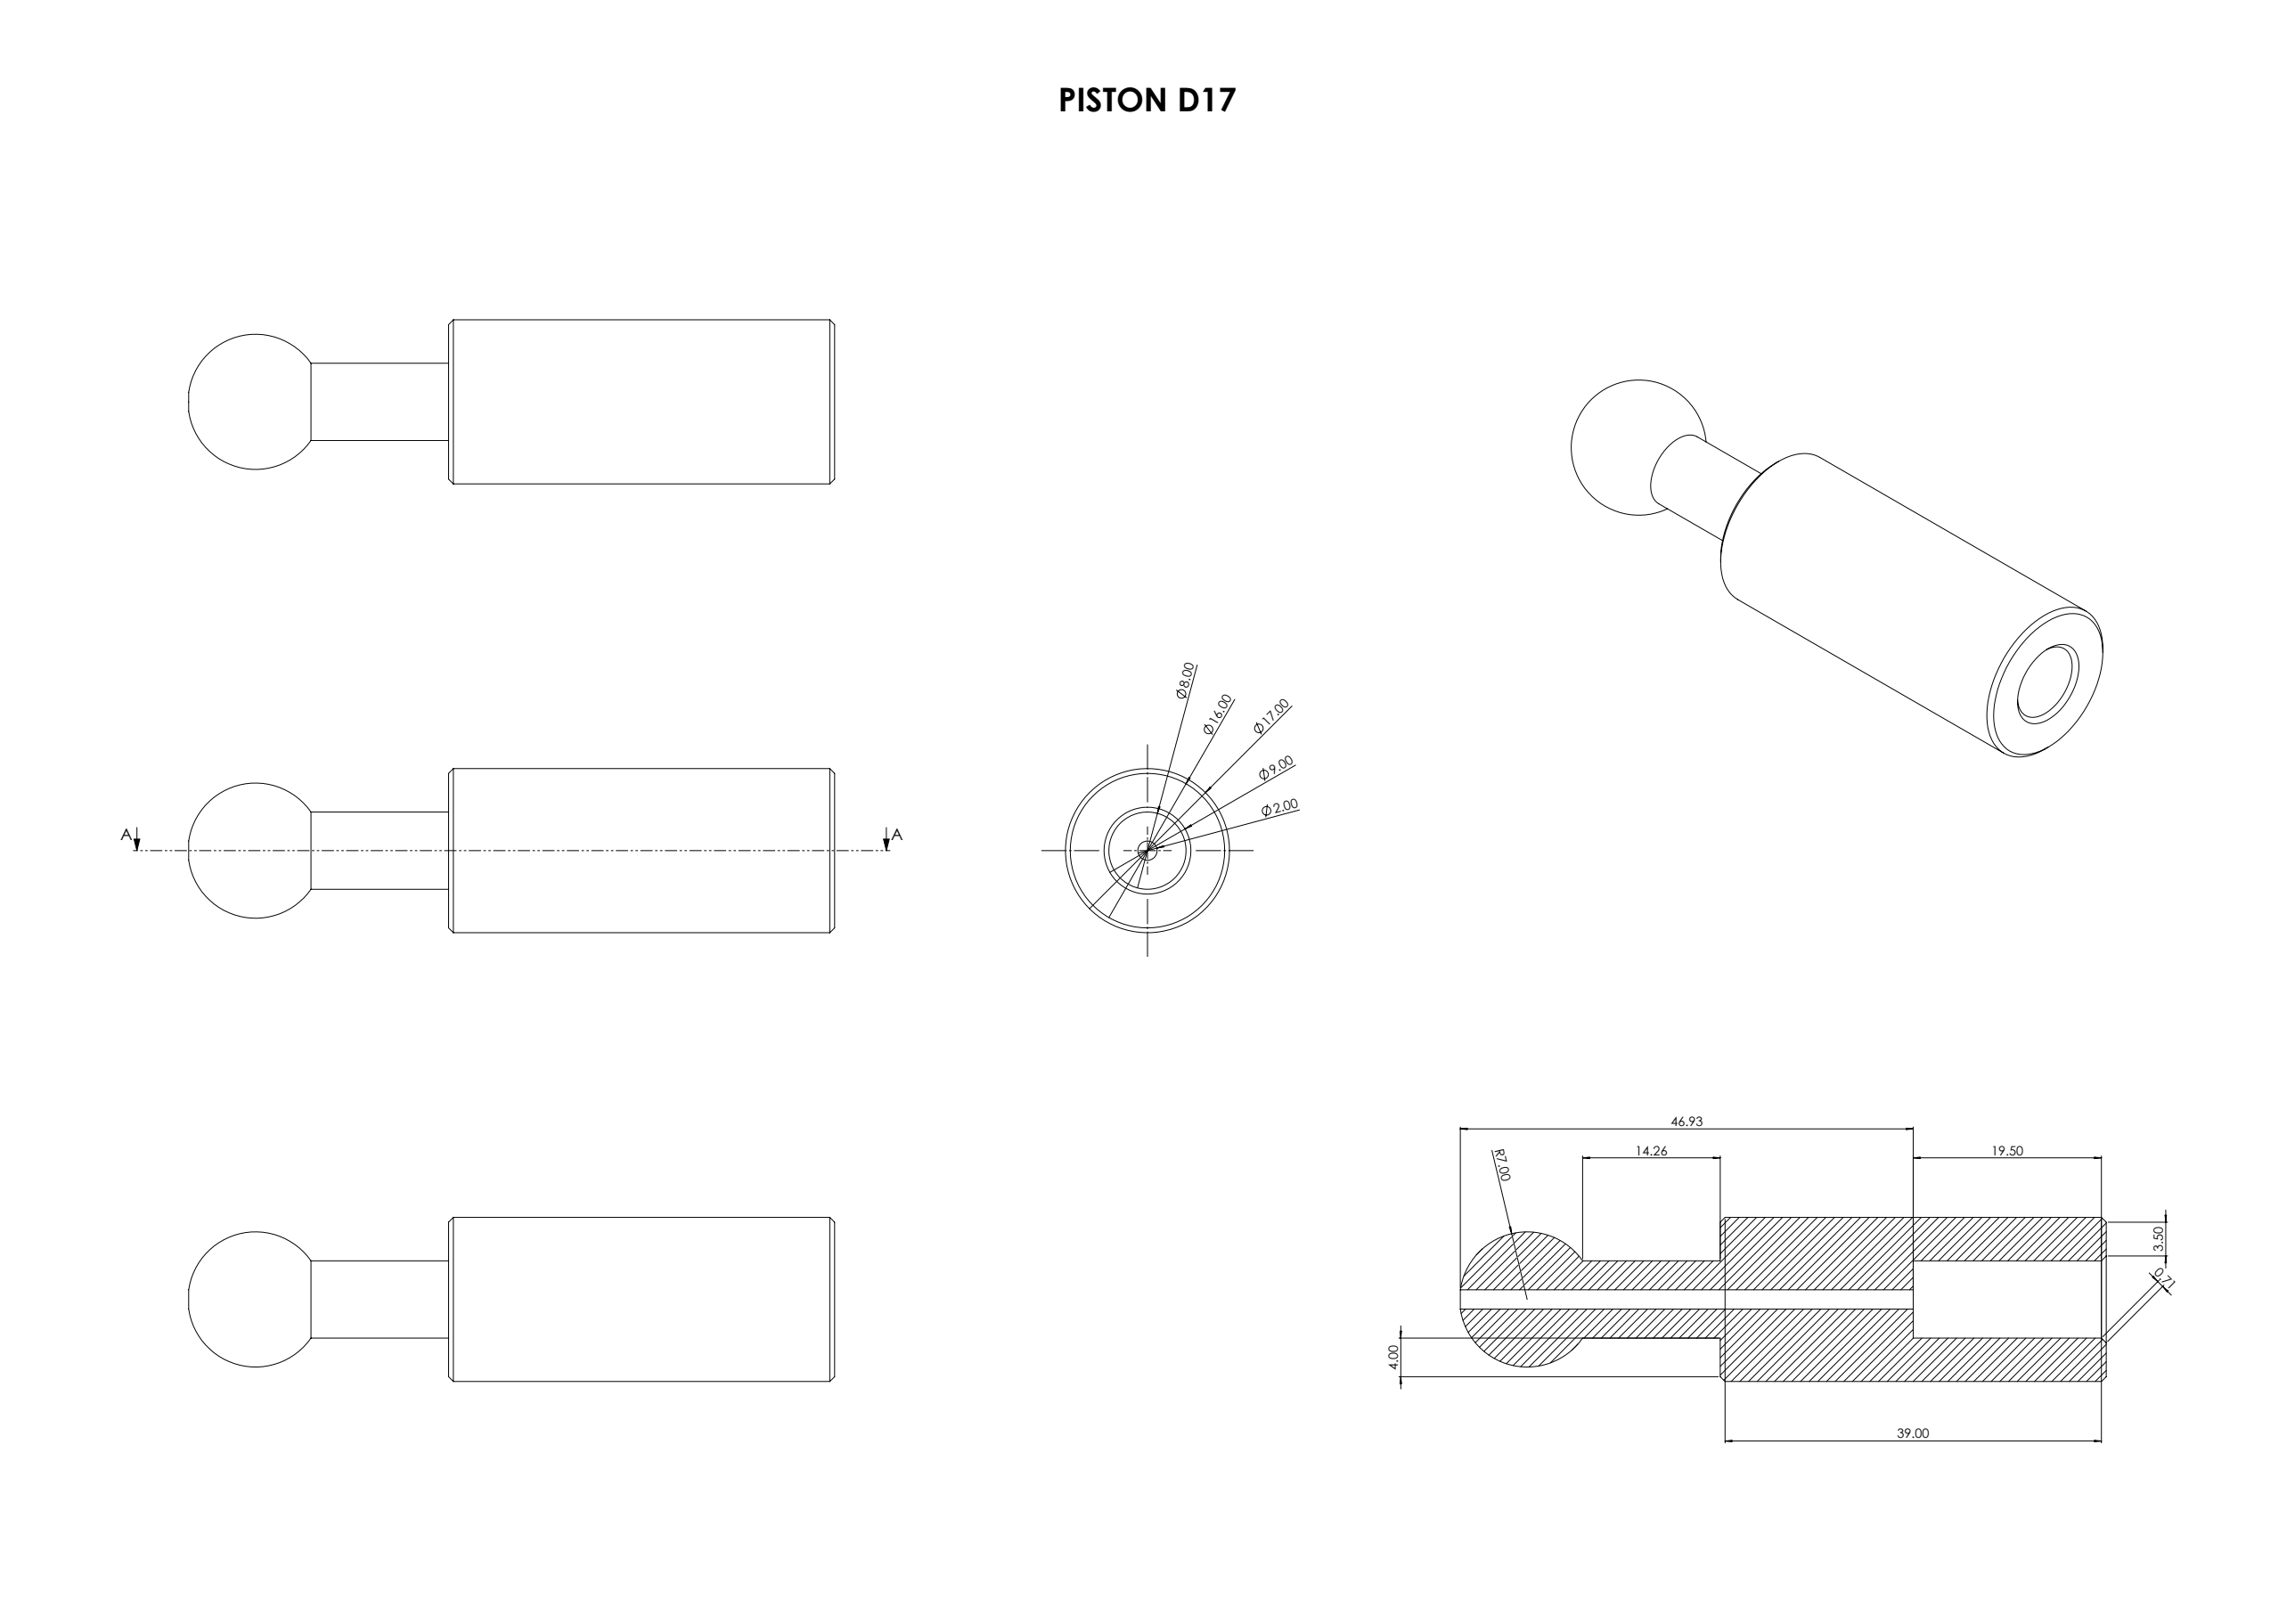
ISO-10303-21;
HEADER;
/* Generated by software containing ST-Developer
 * from STEP Tools, Inc. (www.steptools.com) 
 */

FILE_DESCRIPTION(
/* description */ (''),
/* implementation_level */ '2;1');

FILE_NAME(
/* name */ '05_Piston_D17.step',
/* time_stamp */ '2026-10-26T07:49:00-07:00',
/* author */ (''),
/* organization */ (''),
/* preprocessor_version */ 'ST-DEVELOPER v20.2',
/* originating_system */ 'Autodesk Translation Framework v15.15.0.0',
/* authorisation */ '');

FILE_SCHEMA (('AUTOMOTIVE_DESIGN { 1 0 10303 214 3 1 1 }'));
ENDSEC;

DATA;
#10=MECHANICAL_DESIGN_GEOMETRIC_PRESENTATION_REPRESENTATION('',(#187),#38507);
#131=(
BOUNDED_SURFACE()
B_SPLINE_SURFACE(2,2,((#27036,#27037,#27038,#27039,#27040,#27041,#27042,
#27043,#27044),(#27045,#27046,#27047,#27048,#27049,#27050,#27051,#27052,
#27053),(#27054,#27055,#27056,#27057,#27058,#27059,#27060,#27061,#27062),
(#27063,#27064,#27065,#27066,#27067,#27068,#27069,#27070,#27071),(#27072,
#27073,#27074,#27075,#27076,#27077,#27078,#27079,#27080)),.UNSPECIFIED.,
 .F.,.T.,.F.)
B_SPLINE_SURFACE_WITH_KNOTS((3,2,3),(3,2,2,2,3),(-1.42752879197468,-0.232447556257835,
0.962633679459007),(-3.14159265358979,-1.5707963267949,0.,1.5707963267949,
3.14159265358979),.UNSPECIFIED.)
GEOMETRIC_REPRESENTATION_ITEM()
RATIONAL_B_SPLINE_SURFACE(((1.,0.707106781186548,1.,0.707106781186548,1.,
0.707106781186548,1.,0.707106781186548,1.),(0.826721789080264,0.584580583213329,
0.826721789080264,0.584580583213329,0.826721789080264,0.584580583213329,
0.826721789080264,0.584580583213329,0.826721789080264),(1.,0.707106781186548,
1.,0.707106781186548,1.,0.707106781186548,1.,0.707106781186548,1.),(0.826721789080262,
0.584580583213328,0.826721789080262,0.584580583213328,0.826721789080262,
0.584580583213328,0.826721789080262,0.584580583213328,0.826721789080262),
(1.,0.707106781186548,1.,0.707106781186548,1.,0.707106781186548,1.,0.707106781186548,
1.)))
REPRESENTATION_ITEM('')
SURFACE()
);
#157=SHAPE_REPRESENTATION_RELATIONSHIP('SRR','None',#38585,#172);
#172=ADVANCED_BREP_SHAPE_REPRESENTATION('',(#202),#38502);
#187=STYLED_ITEM('',(#38713),#202);
#202=MANIFOLD_SOLID_BREP('Body1',#15081);
#507=FACE_BOUND('',#3150,.T.);
#508=FACE_BOUND('',#3153,.T.);
#509=FACE_BOUND('',#3156,.T.);
#802=PLANE('',#16260);
#803=PLANE('',#16266);
#804=PLANE('',#16271);
#1505=CYLINDRICAL_SURFACE('',#16258,4.);
#1506=CYLINDRICAL_SURFACE('',#16262,1.);
#1507=CYLINDRICAL_SURFACE('',#16267,4.);
#1508=CYLINDRICAL_SURFACE('',#16275,8.5);
#2170=FACE_OUTER_BOUND('',#3147,.T.);
#2171=FACE_OUTER_BOUND('',#3148,.T.);
#2172=FACE_OUTER_BOUND('',#3149,.T.);
#2173=FACE_OUTER_BOUND('',#3151,.T.);
#2174=FACE_OUTER_BOUND('',#3152,.T.);
#2175=FACE_OUTER_BOUND('',#3154,.T.);
#2176=FACE_OUTER_BOUND('',#3155,.T.);
#2177=FACE_OUTER_BOUND('',#3157,.T.);
#2178=FACE_OUTER_BOUND('',#3158,.T.);
#2179=FACE_OUTER_BOUND('',#3159,.T.);
#2180=FACE_OUTER_BOUND('',#3160,.T.);
#3147=EDGE_LOOP('',(#12485,#12486,#12487,#12488));
#3148=EDGE_LOOP('',(#12489,#12490,#12491,#12492));
#3149=EDGE_LOOP('',(#12493));
#3150=EDGE_LOOP('',(#12494));
#3151=EDGE_LOOP('',(#12495,#12496,#12497,#12498,#12499));
#3152=EDGE_LOOP('',(#12500));
#3153=EDGE_LOOP('',(#12501));
#3154=EDGE_LOOP('',(#12502,#12503,#12504,#12505,#12506));
#3155=EDGE_LOOP('',(#12507));
#3156=EDGE_LOOP('',(#12508));
#3157=EDGE_LOOP('',(#12509,#12510,#12511,#12512));
#3158=EDGE_LOOP('',(#12513,#12514,#12515,#12516));
#3159=EDGE_LOOP('',(#12517,#12518,#12519,#12520));
#3160=EDGE_LOOP('',(#12521,#12522,#12523,#12524,#12525,#12526));
#4129=LINE('',#26997,#5198);
#4130=LINE('',#27002,#5199);
#4131=LINE('',#27011,#5200);
#4132=LINE('',#27019,#5201);
#4133=LINE('',#27029,#5202);
#4134=LINE('',#27033,#5203);
#4135=LINE('',#27035,#5204);
#5198=VECTOR('',#19382,4.25);
#5199=VECTOR('',#19389,4.);
#5200=VECTOR('',#19398,1.);
#5201=VECTOR('',#19409,4.);
#5202=VECTOR('',#19422,8.25);
#5203=VECTOR('',#19427,8.5);
#5204=VECTOR('',#19430,8.25);
#6114=CIRCLE('',#16256,4.5);
#6115=CIRCLE('',#16257,4.);
#6116=CIRCLE('',#16259,4.);
#6117=CIRCLE('',#16261,8.);
#6118=CIRCLE('',#16263,1.);
#6119=CIRCLE('',#16264,1.);
#6120=CIRCLE('',#16265,1.);
#6121=CIRCLE('',#16268,4.);
#6122=CIRCLE('',#16269,4.);
#6123=CIRCLE('',#16270,4.);
#6124=CIRCLE('',#16272,8.);
#6125=CIRCLE('',#16274,8.5);
#6126=CIRCLE('',#16276,8.5);
#6127=CIRCLE('',#16278,6.99981782686978);
#7119=VERTEX_POINT('',#26994);
#7120=VERTEX_POINT('',#26996);
#7121=VERTEX_POINT('',#27000);
#7122=VERTEX_POINT('',#27004);
#7123=VERTEX_POINT('',#27007);
#7124=VERTEX_POINT('',#27008);
#7125=VERTEX_POINT('',#27010);
#7126=VERTEX_POINT('',#27016);
#7127=VERTEX_POINT('',#27018);
#7128=VERTEX_POINT('',#27020);
#7129=VERTEX_POINT('',#27024);
#7130=VERTEX_POINT('',#27027);
#7131=VERTEX_POINT('',#27031);
#8991=EDGE_CURVE('',#7119,#7119,#6114,.T.);
#8992=EDGE_CURVE('',#7119,#7120,#4129,.T.);
#8993=EDGE_CURVE('',#7120,#7120,#6115,.T.);
#8994=EDGE_CURVE('',#7121,#7121,#6116,.T.);
#8995=EDGE_CURVE('',#7121,#7120,#4130,.T.);
#8996=EDGE_CURVE('',#7122,#7122,#6117,.T.);
#8997=EDGE_CURVE('',#7123,#7124,#6118,.T.);
#8998=EDGE_CURVE('',#7123,#7125,#4131,.T.);
#8999=EDGE_CURVE('',#7125,#7125,#6119,.T.);
#9000=EDGE_CURVE('',#7124,#7123,#6120,.T.);
#9001=EDGE_CURVE('',#7126,#7126,#6121,.T.);
#9002=EDGE_CURVE('',#7126,#7127,#4132,.T.);
#9003=EDGE_CURVE('',#7127,#7128,#6122,.T.);
#9004=EDGE_CURVE('',#7128,#7127,#6123,.T.);
#9005=EDGE_CURVE('',#7129,#7129,#6124,.T.);
#9006=EDGE_CURVE('',#7130,#7130,#6125,.T.);
#9007=EDGE_CURVE('',#7130,#7129,#4133,.T.);
#9008=EDGE_CURVE('',#7131,#7131,#6126,.T.);
#9009=EDGE_CURVE('',#7131,#7130,#4134,.T.);
#9010=EDGE_CURVE('',#7122,#7131,#4135,.T.);
#9011=EDGE_CURVE('',#7128,#7124,#6127,.T.);
#12485=ORIENTED_EDGE('',*,*,#8991,.T.);
#12486=ORIENTED_EDGE('',*,*,#8992,.T.);
#12487=ORIENTED_EDGE('',*,*,#8993,.T.);
#12488=ORIENTED_EDGE('',*,*,#8992,.F.);
#12489=ORIENTED_EDGE('',*,*,#8994,.F.);
#12490=ORIENTED_EDGE('',*,*,#8995,.T.);
#12491=ORIENTED_EDGE('',*,*,#8993,.F.);
#12492=ORIENTED_EDGE('',*,*,#8995,.F.);
#12493=ORIENTED_EDGE('',*,*,#8996,.T.);
#12494=ORIENTED_EDGE('',*,*,#8991,.F.);
#12495=ORIENTED_EDGE('',*,*,#8997,.F.);
#12496=ORIENTED_EDGE('',*,*,#8998,.T.);
#12497=ORIENTED_EDGE('',*,*,#8999,.F.);
#12498=ORIENTED_EDGE('',*,*,#8998,.F.);
#12499=ORIENTED_EDGE('',*,*,#9000,.F.);
#12500=ORIENTED_EDGE('',*,*,#8994,.T.);
#12501=ORIENTED_EDGE('',*,*,#8999,.T.);
#12502=ORIENTED_EDGE('',*,*,#9001,.F.);
#12503=ORIENTED_EDGE('',*,*,#9002,.T.);
#12504=ORIENTED_EDGE('',*,*,#9003,.T.);
#12505=ORIENTED_EDGE('',*,*,#9004,.T.);
#12506=ORIENTED_EDGE('',*,*,#9002,.F.);
#12507=ORIENTED_EDGE('',*,*,#9005,.F.);
#12508=ORIENTED_EDGE('',*,*,#9001,.T.);
#12509=ORIENTED_EDGE('',*,*,#9006,.F.);
#12510=ORIENTED_EDGE('',*,*,#9007,.T.);
#12511=ORIENTED_EDGE('',*,*,#9005,.T.);
#12512=ORIENTED_EDGE('',*,*,#9007,.F.);
#12513=ORIENTED_EDGE('',*,*,#9008,.F.);
#12514=ORIENTED_EDGE('',*,*,#9009,.T.);
#12515=ORIENTED_EDGE('',*,*,#9006,.T.);
#12516=ORIENTED_EDGE('',*,*,#9009,.F.);
#12517=ORIENTED_EDGE('',*,*,#8996,.F.);
#12518=ORIENTED_EDGE('',*,*,#9010,.T.);
#12519=ORIENTED_EDGE('',*,*,#9008,.T.);
#12520=ORIENTED_EDGE('',*,*,#9010,.F.);
#12521=ORIENTED_EDGE('',*,*,#9003,.F.);
#12522=ORIENTED_EDGE('',*,*,#9004,.F.);
#12523=ORIENTED_EDGE('',*,*,#9011,.T.);
#12524=ORIENTED_EDGE('',*,*,#9000,.T.);
#12525=ORIENTED_EDGE('',*,*,#8997,.T.);
#12526=ORIENTED_EDGE('',*,*,#9011,.F.);
#14175=CONICAL_SURFACE('',#16255,4.25,0.78539816339745);
#14176=CONICAL_SURFACE('',#16273,8.25,0.78539816339745);
#14177=CONICAL_SURFACE('',#16277,8.25,0.78539816339745);
#14737=ADVANCED_FACE('',(#2170),#14175,.F.);
#14738=ADVANCED_FACE('',(#2171),#1505,.F.);
#14739=ADVANCED_FACE('',(#2172,#507),#802,.T.);
#14740=ADVANCED_FACE('',(#2173),#1506,.F.);
#14741=ADVANCED_FACE('',(#2174,#508),#803,.F.);
#14742=ADVANCED_FACE('',(#2175),#1507,.T.);
#14743=ADVANCED_FACE('',(#2176,#509),#804,.T.);
#14744=ADVANCED_FACE('',(#2177),#14176,.T.);
#14745=ADVANCED_FACE('',(#2178),#1508,.T.);
#14746=ADVANCED_FACE('',(#2179),#14177,.T.);
#14747=ADVANCED_FACE('',(#2180),#131,.F.);
#15081=CLOSED_SHELL('',(#14737,#14738,#14739,#14740,#14741,#14742,#14743,
#14744,#14745,#14746,#14747));
#16254=AXIS2_PLACEMENT_3D('',#26992,#19376,#19377);
#16255=AXIS2_PLACEMENT_3D('',#26993,#19378,#19379);
#16256=AXIS2_PLACEMENT_3D('',#26995,#19380,#19381);
#16257=AXIS2_PLACEMENT_3D('',#26998,#19383,#19384);
#16258=AXIS2_PLACEMENT_3D('',#26999,#19385,#19386);
#16259=AXIS2_PLACEMENT_3D('',#27001,#19387,#19388);
#16260=AXIS2_PLACEMENT_3D('',#27003,#19390,#19391);
#16261=AXIS2_PLACEMENT_3D('',#27005,#19392,#19393);
#16262=AXIS2_PLACEMENT_3D('',#27006,#19394,#19395);
#16263=AXIS2_PLACEMENT_3D('',#27009,#19396,#19397);
#16264=AXIS2_PLACEMENT_3D('',#27012,#19399,#19400);
#16265=AXIS2_PLACEMENT_3D('',#27013,#19401,#19402);
#16266=AXIS2_PLACEMENT_3D('',#27014,#19403,#19404);
#16267=AXIS2_PLACEMENT_3D('',#27015,#19405,#19406);
#16268=AXIS2_PLACEMENT_3D('',#27017,#19407,#19408);
#16269=AXIS2_PLACEMENT_3D('',#27021,#19410,#19411);
#16270=AXIS2_PLACEMENT_3D('',#27022,#19412,#19413);
#16271=AXIS2_PLACEMENT_3D('',#27023,#19414,#19415);
#16272=AXIS2_PLACEMENT_3D('',#27025,#19416,#19417);
#16273=AXIS2_PLACEMENT_3D('',#27026,#19418,#19419);
#16274=AXIS2_PLACEMENT_3D('',#27028,#19420,#19421);
#16275=AXIS2_PLACEMENT_3D('',#27030,#19423,#19424);
#16276=AXIS2_PLACEMENT_3D('',#27032,#19425,#19426);
#16277=AXIS2_PLACEMENT_3D('',#27034,#19428,#19429);
#16278=AXIS2_PLACEMENT_3D('',#27081,#19431,#19432);
#19376=DIRECTION('axis',(0.,0.,1.));
#19377=DIRECTION('refdir',(1.,0.,0.));
#19378=DIRECTION('center_axis',(1.,0.,0.));
#19379=DIRECTION('ref_axis',(0.,1.,0.));
#19380=DIRECTION('center_axis',(1.,0.,0.));
#19381=DIRECTION('ref_axis',(0.,1.,0.));
#19382=DIRECTION('',(-0.707106781186546,0.707106781186549,8.65956056235495E-17));
#19383=DIRECTION('center_axis',(-1.,0.,0.));
#19384=DIRECTION('ref_axis',(0.,1.,0.));
#19385=DIRECTION('center_axis',(1.,0.,0.));
#19386=DIRECTION('ref_axis',(0.,1.,0.));
#19387=DIRECTION('center_axis',(1.,0.,0.));
#19388=DIRECTION('ref_axis',(0.,0.,-1.));
#19389=DIRECTION('',(1.,0.,0.));
#19390=DIRECTION('center_axis',(1.,0.,0.));
#19391=DIRECTION('ref_axis',(0.,0.,-1.));
#19392=DIRECTION('center_axis',(1.,0.,0.));
#19393=DIRECTION('ref_axis',(0.,0.,-1.));
#19394=DIRECTION('center_axis',(1.,0.,0.));
#19395=DIRECTION('ref_axis',(0.,1.,0.));
#19396=DIRECTION('center_axis',(1.,0.,0.));
#19397=DIRECTION('ref_axis',(0.,1.,0.));
#19398=DIRECTION('',(1.,0.,0.));
#19399=DIRECTION('center_axis',(-1.,0.,0.));
#19400=DIRECTION('ref_axis',(0.,1.,0.));
#19401=DIRECTION('center_axis',(1.,0.,0.));
#19402=DIRECTION('ref_axis',(0.,1.,0.));
#19403=DIRECTION('center_axis',(-1.,0.,0.));
#19404=DIRECTION('ref_axis',(0.,0.,1.));
#19405=DIRECTION('center_axis',(1.,0.,0.));
#19406=DIRECTION('ref_axis',(0.,1.,0.));
#19407=DIRECTION('center_axis',(1.,0.,0.));
#19408=DIRECTION('ref_axis',(0.,0.,-1.));
#19409=DIRECTION('',(-1.,0.,0.));
#19410=DIRECTION('center_axis',(1.,0.,0.));
#19411=DIRECTION('ref_axis',(0.,0.,-1.));
#19412=DIRECTION('center_axis',(1.,0.,0.));
#19413=DIRECTION('ref_axis',(0.,0.,-1.));
#19414=DIRECTION('center_axis',(-1.,0.,0.));
#19415=DIRECTION('ref_axis',(0.,0.,1.));
#19416=DIRECTION('center_axis',(1.,0.,0.));
#19417=DIRECTION('ref_axis',(0.,0.,-1.));
#19418=DIRECTION('center_axis',(1.,0.,0.));
#19419=DIRECTION('ref_axis',(0.,1.,0.));
#19420=DIRECTION('center_axis',(1.,0.,0.));
#19421=DIRECTION('ref_axis',(0.,0.,-1.));
#19422=DIRECTION('',(-0.707106781186547,0.707106781186548,8.65956056235494E-17));
#19423=DIRECTION('center_axis',(1.,0.,0.));
#19424=DIRECTION('ref_axis',(0.,1.,0.));
#19425=DIRECTION('center_axis',(1.,0.,0.));
#19426=DIRECTION('ref_axis',(0.,0.,-1.));
#19427=DIRECTION('',(-1.,0.,0.));
#19428=DIRECTION('center_axis',(-1.,0.,0.));
#19429=DIRECTION('ref_axis',(0.,1.,0.));
#19430=DIRECTION('',(-0.707106781186547,-0.707106781186548,-8.65956056235494E-17));
#19431=DIRECTION('center_axis',(0.,-1.,-1.22464679914735E-16));
#19432=DIRECTION('ref_axis',(0.,-1.22464679914735E-16,1.));
#26992=CARTESIAN_POINT('',(0.,0.,0.));
#26993=CARTESIAN_POINT('Origin',(59.75,0.,0.));
#26994=CARTESIAN_POINT('',(60.,-4.5,-5.51091059616309E-16));
#26995=CARTESIAN_POINT('Origin',(60.,0.,0.));
#26996=CARTESIAN_POINT('',(59.5,-4.,4.89858719658941E-16));
#26997=CARTESIAN_POINT('',(59.75,-4.25,-5.20474889637625E-16));
#26998=CARTESIAN_POINT('Origin',(59.5,0.,0.));
#26999=CARTESIAN_POINT('Origin',(50.05,0.,0.));
#27000=CARTESIAN_POINT('',(40.,-4.,-4.89858719658941E-16));
#27001=CARTESIAN_POINT('Origin',(40.,0.,0.));
#27002=CARTESIAN_POINT('',(50.05,-4.,-4.89858719658941E-16));
#27003=CARTESIAN_POINT('Origin',(60.,0.,0.));
#27004=CARTESIAN_POINT('',(60.,-8.,-9.79717439317882E-16));
#27005=CARTESIAN_POINT('Origin',(60.,0.,0.));
#27006=CARTESIAN_POINT('Origin',(26.5,0.,0.));
#27007=CARTESIAN_POINT('',(-6.92828513265203,-1.,-1.22464679914735E-16));
#27008=CARTESIAN_POINT('',(-6.92828513265203,-1.22464679914735E-16,1.));
#27009=CARTESIAN_POINT('Origin',(-6.92828513265203,0.,0.));
#27010=CARTESIAN_POINT('',(40.,-1.,1.22464679914735E-16));
#27011=CARTESIAN_POINT('',(26.5,-1.,-1.22464679914735E-16));
#27012=CARTESIAN_POINT('Origin',(40.,0.,0.));
#27013=CARTESIAN_POINT('Origin',(-6.92828513265203,0.,0.));
#27014=CARTESIAN_POINT('Origin',(40.,4.,0.));
#27015=CARTESIAN_POINT('Origin',(12.872281323269,0.,0.));
#27016=CARTESIAN_POINT('',(20.,-4.,-4.89858719658941E-16));
#27017=CARTESIAN_POINT('Origin',(20.,0.,0.));
#27018=CARTESIAN_POINT('',(5.74456264653803,-4.,-4.89858719658941E-16));
#27019=CARTESIAN_POINT('',(12.872281323269,-4.,-4.89858719658941E-16));
#27020=CARTESIAN_POINT('',(5.74456264653803,-4.89858719658941E-16,4.));
#27021=CARTESIAN_POINT('Origin',(5.74456264653803,0.,0.));
#27022=CARTESIAN_POINT('Origin',(5.74456264653803,0.,0.));
#27023=CARTESIAN_POINT('Origin',(20.,8.,0.));
#27024=CARTESIAN_POINT('',(20.,-8.,-9.79717439317883E-16));
#27025=CARTESIAN_POINT('Origin',(20.,0.,0.));
#27026=CARTESIAN_POINT('Origin',(20.25,0.,0.));
#27027=CARTESIAN_POINT('',(20.5,-8.5,-1.04094977927525E-15));
#27028=CARTESIAN_POINT('Origin',(20.5,0.,0.));
#27029=CARTESIAN_POINT('',(20.25,-8.25,-1.01033360929657E-15));
#27030=CARTESIAN_POINT('Origin',(40.,0.,0.));
#27031=CARTESIAN_POINT('',(59.5,-8.5,-1.04094977927525E-15));
#27032=CARTESIAN_POINT('Origin',(59.5,0.,0.));
#27033=CARTESIAN_POINT('',(40.,-8.5,-1.04094977927525E-15));
#27034=CARTESIAN_POINT('Origin',(59.75,0.,0.));
#27035=CARTESIAN_POINT('',(59.75,-8.25,-1.01033360929657E-15));
#27036=CARTESIAN_POINT('Ctrl Pts',(-6.92828513265203,0.,1.));
#27037=CARTESIAN_POINT('Ctrl Pts',(-6.92828513265203,-1.,1.));
#27038=CARTESIAN_POINT('Ctrl Pts',(-6.92828513265203,-1.,0.));
#27039=CARTESIAN_POINT('Ctrl Pts',(-6.92828513265203,-1.,-1.));
#27040=CARTESIAN_POINT('Ctrl Pts',(-6.92828513265203,0.,-1.));
#27041=CARTESIAN_POINT('Ctrl Pts',(-6.92828513265203,1.,-1.));
#27042=CARTESIAN_POINT('Ctrl Pts',(-6.92828513265203,1.,0.));
#27043=CARTESIAN_POINT('Ctrl Pts',(-6.92828513265203,1.,1.));
#27044=CARTESIAN_POINT('Ctrl Pts',(-6.92828513265203,0.,1.));
#27045=CARTESIAN_POINT('Ctrl Pts',(-6.24814779917882,0.,5.71479842490333));
#27046=CARTESIAN_POINT('Ctrl Pts',(-6.24814779917882,-5.71479842490333,
5.71479842490333));
#27047=CARTESIAN_POINT('Ctrl Pts',(-6.24814779917882,-5.71479842490333,
0.));
#27048=CARTESIAN_POINT('Ctrl Pts',(-6.24814779917882,-5.71479842490333,
-5.71479842490333));
#27049=CARTESIAN_POINT('Ctrl Pts',(-6.24814779917882,0.,-5.71479842490333));
#27050=CARTESIAN_POINT('Ctrl Pts',(-6.24814779917882,5.71479842490333,-5.71479842490333));
#27051=CARTESIAN_POINT('Ctrl Pts',(-6.24814779917882,5.71479842490333,0.));
#27052=CARTESIAN_POINT('Ctrl Pts',(-6.24814779917882,5.71479842490333,5.71479842490333));
#27053=CARTESIAN_POINT('Ctrl Pts',(-6.24814779917882,0.,5.71479842490333));
#27054=CARTESIAN_POINT('Ctrl Pts',(-1.61265982287702,0.,6.81214167175753));
#27055=CARTESIAN_POINT('Ctrl Pts',(-1.61265982287702,-6.81214167175752,
6.81214167175752));
#27056=CARTESIAN_POINT('Ctrl Pts',(-1.61265982287702,-6.81214167175753,
0.));
#27057=CARTESIAN_POINT('Ctrl Pts',(-1.61265982287702,-6.81214167175752,
-6.81214167175752));
#27058=CARTESIAN_POINT('Ctrl Pts',(-1.61265982287702,0.,-6.81214167175753));
#27059=CARTESIAN_POINT('Ctrl Pts',(-1.61265982287702,6.81214167175752,-6.81214167175752));
#27060=CARTESIAN_POINT('Ctrl Pts',(-1.61265982287702,6.81214167175753,0.));
#27061=CARTESIAN_POINT('Ctrl Pts',(-1.61265982287702,6.81214167175752,6.81214167175752));
#27062=CARTESIAN_POINT('Ctrl Pts',(-1.61265982287702,0.,6.81214167175753));
#27063=CARTESIAN_POINT('Ctrl Pts',(3.02282815342477,0.,7.90948491861172));
#27064=CARTESIAN_POINT('Ctrl Pts',(3.02282815342477,-7.90948491861172,7.90948491861172));
#27065=CARTESIAN_POINT('Ctrl Pts',(3.02282815342477,-7.90948491861172,0.));
#27066=CARTESIAN_POINT('Ctrl Pts',(3.02282815342477,-7.90948491861172,-7.90948491861172));
#27067=CARTESIAN_POINT('Ctrl Pts',(3.02282815342477,0.,-7.90948491861172));
#27068=CARTESIAN_POINT('Ctrl Pts',(3.02282815342477,7.90948491861172,-7.90948491861172));
#27069=CARTESIAN_POINT('Ctrl Pts',(3.02282815342477,7.90948491861172,0.));
#27070=CARTESIAN_POINT('Ctrl Pts',(3.02282815342477,7.90948491861172,7.90948491861172));
#27071=CARTESIAN_POINT('Ctrl Pts',(3.02282815342477,0.,7.90948491861172));
#27072=CARTESIAN_POINT('Ctrl Pts',(5.74456264653803,0.,4.));
#27073=CARTESIAN_POINT('Ctrl Pts',(5.74456264653803,-4.,4.));
#27074=CARTESIAN_POINT('Ctrl Pts',(5.74456264653803,-4.,0.));
#27075=CARTESIAN_POINT('Ctrl Pts',(5.74456264653803,-4.,-4.));
#27076=CARTESIAN_POINT('Ctrl Pts',(5.74456264653803,0.,-4.));
#27077=CARTESIAN_POINT('Ctrl Pts',(5.74456264653803,4.,-4.));
#27078=CARTESIAN_POINT('Ctrl Pts',(5.74456264653803,4.,0.));
#27079=CARTESIAN_POINT('Ctrl Pts',(5.74456264653803,4.,4.));
#27080=CARTESIAN_POINT('Ctrl Pts',(5.74456264653803,0.,4.));
#27081=CARTESIAN_POINT('Origin',(-0.000182197201354928,-7.10914706616621E-20,
0.000580505911673135));
#38485=UNCERTAINTY_MEASURE_WITH_UNIT(LENGTH_MEASURE(0.01),#38508,
'DISTANCE_ACCURACY_VALUE',
'Maximum model space distance between geometric entities at asserted c
onnectivities');
#38490=UNCERTAINTY_MEASURE_WITH_UNIT(LENGTH_MEASURE(0.01),#38508,
'DISTANCE_ACCURACY_VALUE',
'Maximum model space distance between geometric entities at asserted c
onnectivities');
#38502=(
GEOMETRIC_REPRESENTATION_CONTEXT(3)
GLOBAL_UNCERTAINTY_ASSIGNED_CONTEXT((#38485))
GLOBAL_UNIT_ASSIGNED_CONTEXT((#38508,#38510,#38511))
REPRESENTATION_CONTEXT('','3D')
);
#38507=(
GEOMETRIC_REPRESENTATION_CONTEXT(3)
GLOBAL_UNCERTAINTY_ASSIGNED_CONTEXT((#38490))
GLOBAL_UNIT_ASSIGNED_CONTEXT((#38508,#38510,#38511))
REPRESENTATION_CONTEXT('','3D')
);
#38508=(
LENGTH_UNIT()
NAMED_UNIT(*)
SI_UNIT(.MILLI.,.METRE.)
);
#38510=(
NAMED_UNIT(*)
PLANE_ANGLE_UNIT()
SI_UNIT($,.RADIAN.)
);
#38511=(
NAMED_UNIT(*)
SI_UNIT($,.STERADIAN.)
SOLID_ANGLE_UNIT()
);
#38523=SHAPE_DEFINITION_REPRESENTATION(#38539,#38585);
#38539=PRODUCT_DEFINITION_SHAPE('',$,#38602);
#38585=SHAPE_REPRESENTATION('',(#16254),#38502);
#38590=PRODUCT_DEFINITION_CONTEXT('part definition',#38640,'design');
#38602=PRODUCT_DEFINITION('2026-10-26-01-10-48-079','05_Piston_D17',#38618,
#38590);
#38618=PRODUCT_DEFINITION_FORMATION('',$,#38653);
#38640=APPLICATION_CONTEXT(
'Core Data for Automotive Mechanical Design Process');
#38641=PRODUCT_CONTEXT('part definition',#38640,'mechanical');
#38653=PRODUCT('2026-10-26-01-10-48-079','05_Piston_D17',$,(#38641));
#38707=COLOUR_RGB('Sky Blue',0.24,0.69,0.87);
#38708=FILL_AREA_STYLE_COLOUR('',#38707);
#38709=FILL_AREA_STYLE('',(#38708));
#38710=SURFACE_STYLE_FILL_AREA(#38709);
#38711=SURFACE_SIDE_STYLE('',(#38710));
#38712=SURFACE_STYLE_USAGE(.BOTH.,#38711);
#38713=PRESENTATION_STYLE_ASSIGNMENT((#38712));
ENDSEC;
END-ISO-10303-21;
